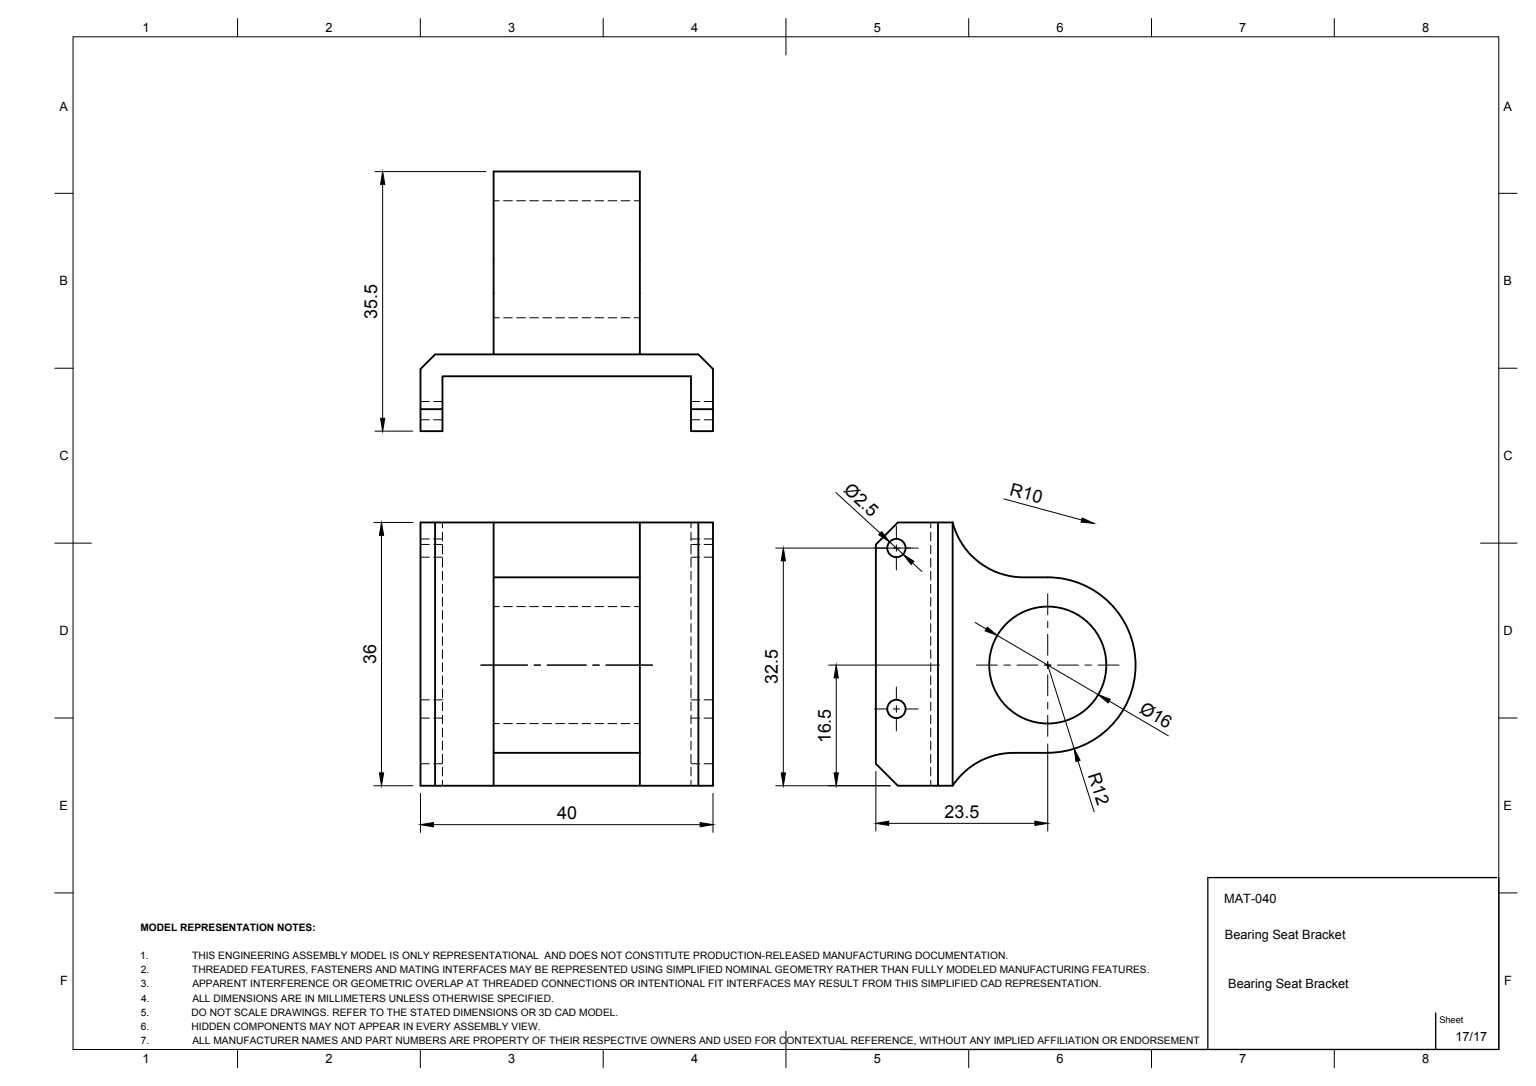
ISO-10303-21;
HEADER;
/* Generated by software containing ST-Developer
 * from STEP Tools, Inc. (www.steptools.com) 
 */

FILE_DESCRIPTION(
/* description */ ('STEP AP214'),
/* implementation_level */ '2;1');

FILE_NAME(
/* name */ 'Bearing Seat Bracket.step',
/* time_stamp */ '2026-11-14T21:53:28-08:00',
/* author */ (''),
/* organization */ (''),
/* preprocessor_version */ 'ST-DEVELOPER v20.2',
/* originating_system */ 'Autodesk Translation Framework v15.17.0.0',
/* authorisation */ '');

FILE_SCHEMA (('AUTOMOTIVE_DESIGN { 1 0 10303 214 3 1 1 }'));
ENDSEC;

DATA;
#10=MECHANICAL_DESIGN_GEOMETRIC_PRESENTATION_REPRESENTATION('',(#332),#20176);
#300=SHAPE_REPRESENTATION_RELATIONSHIP('SRR','None',#20264,#312);
#312=ADVANCED_BREP_SHAPE_REPRESENTATION('',(#359),#20170);
#332=STYLED_ITEM('',(#20338),#359);
#359=MANIFOLD_SOLID_BREP('Body1',#10950);
#546=FACE_BOUND('',#2149,.T.);
#547=FACE_BOUND('',#2150,.T.);
#548=FACE_BOUND('',#2153,.T.);
#549=FACE_BOUND('',#2154,.T.);
#550=FACE_BOUND('',#2157,.T.);
#551=FACE_BOUND('',#2158,.T.);
#552=FACE_BOUND('',#2160,.T.);
#553=FACE_BOUND('',#2161,.T.);
#554=FACE_BOUND('',#2174,.T.);
#555=FACE_BOUND('',#2177,.T.);
#846=PLANE('',#11980);
#847=PLANE('',#11981);
#848=PLANE('',#11982);
#849=PLANE('',#11983);
#850=PLANE('',#11984);
#851=PLANE('',#11985);
#852=PLANE('',#11986);
#853=PLANE('',#11987);
#854=PLANE('',#11988);
#855=PLANE('',#11989);
#856=PLANE('',#11990);
#857=PLANE('',#11991);
#858=PLANE('',#11992);
#859=PLANE('',#11996);
#860=PLANE('',#11997);
#861=PLANE('',#12004);
#862=PLANE('',#12005);
#863=PLANE('',#12006);
#864=PLANE('',#12007);
#865=PLANE('',#12008);
#866=PLANE('',#12009);
#1384=FACE_OUTER_BOUND('',#2142,.T.);
#1385=FACE_OUTER_BOUND('',#2143,.T.);
#1386=FACE_OUTER_BOUND('',#2144,.T.);
#1387=FACE_OUTER_BOUND('',#2145,.T.);
#1388=FACE_OUTER_BOUND('',#2146,.T.);
#1389=FACE_OUTER_BOUND('',#2147,.T.);
#1390=FACE_OUTER_BOUND('',#2148,.T.);
#1391=FACE_OUTER_BOUND('',#2151,.T.);
#1392=FACE_OUTER_BOUND('',#2152,.T.);
#1393=FACE_OUTER_BOUND('',#2155,.T.);
#1394=FACE_OUTER_BOUND('',#2156,.T.);
#1395=FACE_OUTER_BOUND('',#2159,.T.);
#1396=FACE_OUTER_BOUND('',#2162,.T.);
#1397=FACE_OUTER_BOUND('',#2163,.T.);
#1398=FACE_OUTER_BOUND('',#2164,.T.);
#1399=FACE_OUTER_BOUND('',#2165,.T.);
#1400=FACE_OUTER_BOUND('',#2166,.T.);
#1401=FACE_OUTER_BOUND('',#2167,.T.);
#1402=FACE_OUTER_BOUND('',#2168,.T.);
#1403=FACE_OUTER_BOUND('',#2169,.T.);
#1404=FACE_OUTER_BOUND('',#2170,.T.);
#1405=FACE_OUTER_BOUND('',#2171,.T.);
#1406=FACE_OUTER_BOUND('',#2172,.T.);
#1407=FACE_OUTER_BOUND('',#2173,.T.);
#1408=FACE_OUTER_BOUND('',#2175,.T.);
#1409=FACE_OUTER_BOUND('',#2176,.T.);
#1410=FACE_OUTER_BOUND('',#2178,.T.);
#1411=FACE_OUTER_BOUND('',#2179,.T.);
#1412=FACE_OUTER_BOUND('',#2180,.T.);
#2142=EDGE_LOOP('',(#9717,#9718,#9719,#9720));
#2143=EDGE_LOOP('',(#9721,#9722,#9723,#9724));
#2144=EDGE_LOOP('',(#9725,#9726,#9727,#9728));
#2145=EDGE_LOOP('',(#9729,#9730,#9731,#9732));
#2146=EDGE_LOOP('',(#9733,#9734,#9735,#9736));
#2147=EDGE_LOOP('',(#9737,#9738,#9739,#9740));
#2148=EDGE_LOOP('',(#9741,#9742,#9743,#9744,#9745,#9746));
#2149=EDGE_LOOP('',(#9747));
#2150=EDGE_LOOP('',(#9748));
#2151=EDGE_LOOP('',(#9749,#9750,#9751,#9752));
#2152=EDGE_LOOP('',(#9753,#9754,#9755,#9756,#9757,#9758));
#2153=EDGE_LOOP('',(#9759));
#2154=EDGE_LOOP('',(#9760));
#2155=EDGE_LOOP('',(#9761,#9762,#9763,#9764));
#2156=EDGE_LOOP('',(#9765,#9766,#9767,#9768,#9769,#9770));
#2157=EDGE_LOOP('',(#9771));
#2158=EDGE_LOOP('',(#9772));
#2159=EDGE_LOOP('',(#9773,#9774,#9775,#9776,#9777,#9778));
#2160=EDGE_LOOP('',(#9779));
#2161=EDGE_LOOP('',(#9780));
#2162=EDGE_LOOP('',(#9781,#9782,#9783,#9784,#9785,#9786,#9787,#9788,#9789,
#9790,#9791,#9792));
#2163=EDGE_LOOP('',(#9793,#9794,#9795,#9796,#9797,#9798,#9799,#9800,#9801,
#9802,#9803,#9804));
#2164=EDGE_LOOP('',(#9805,#9806,#9807,#9808));
#2165=EDGE_LOOP('',(#9809,#9810,#9811,#9812));
#2166=EDGE_LOOP('',(#9813,#9814,#9815,#9816));
#2167=EDGE_LOOP('',(#9817,#9818,#9819,#9820));
#2168=EDGE_LOOP('',(#9821,#9822,#9823,#9824));
#2169=EDGE_LOOP('',(#9825,#9826,#9827,#9828));
#2170=EDGE_LOOP('',(#9829,#9830,#9831,#9832));
#2171=EDGE_LOOP('',(#9833,#9834,#9835,#9836));
#2172=EDGE_LOOP('',(#9837,#9838,#9839,#9840));
#2173=EDGE_LOOP('',(#9841,#9842,#9843,#9844,#9845,#9846));
#2174=EDGE_LOOP('',(#9847));
#2175=EDGE_LOOP('',(#9848,#9849,#9850,#9851));
#2176=EDGE_LOOP('',(#9852,#9853,#9854,#9855,#9856,#9857));
#2177=EDGE_LOOP('',(#9858));
#2178=EDGE_LOOP('',(#9859,#9860,#9861,#9862));
#2179=EDGE_LOOP('',(#9863,#9864,#9865,#9866));
#2180=EDGE_LOOP('',(#9867,#9868,#9869,#9870));
#3146=LINE('',#19626,#4134);
#3147=LINE('',#19632,#4135);
#3148=LINE('',#19638,#4136);
#3149=LINE('',#19644,#4137);
#3150=LINE('',#19650,#4138);
#3151=LINE('',#19655,#4139);
#3152=LINE('',#19657,#4140);
#3153=LINE('',#19659,#4141);
#3154=LINE('',#19660,#4142);
#3155=LINE('',#19664,#4143);
#3156=LINE('',#19665,#4144);
#3157=LINE('',#19667,#4145);
#3158=LINE('',#19669,#4146);
#3159=LINE('',#19670,#4147);
#3160=LINE('',#19673,#4148);
#3161=LINE('',#19675,#4149);
#3162=LINE('',#19676,#4150);
#3163=LINE('',#19680,#4151);
#3164=LINE('',#19682,#4152);
#3165=LINE('',#19683,#4153);
#3166=LINE('',#19685,#4154);
#3167=LINE('',#19686,#4155);
#3168=LINE('',#19690,#4156);
#3169=LINE('',#19691,#4157);
#3170=LINE('',#19692,#4158);
#3171=LINE('',#19696,#4159);
#3172=LINE('',#19698,#4160);
#3173=LINE('',#19700,#4161);
#3174=LINE('',#19701,#4162);
#3175=LINE('',#19702,#4163);
#3176=LINE('',#19706,#4164);
#3177=LINE('',#19708,#4165);
#3178=LINE('',#19710,#4166);
#3179=LINE('',#19711,#4167);
#3180=LINE('',#19712,#4168);
#3181=LINE('',#19715,#4169);
#3182=LINE('',#19717,#4170);
#3183=LINE('',#19719,#4171);
#3184=LINE('',#19721,#4172);
#3185=LINE('',#19722,#4173);
#3186=LINE('',#19723,#4174);
#3187=LINE('',#19724,#4175);
#3188=LINE('',#19728,#4176);
#3189=LINE('',#19729,#4177);
#3190=LINE('',#19730,#4178);
#3191=LINE('',#19731,#4179);
#3192=LINE('',#19733,#4180);
#3193=LINE('',#19735,#4181);
#3194=LINE('',#19736,#4182);
#3195=LINE('',#19746,#4183);
#3196=LINE('',#19749,#4184);
#3197=LINE('',#19752,#4185);
#3198=LINE('',#19754,#4186);
#3199=LINE('',#19755,#4187);
#3200=LINE('',#19758,#4188);
#3201=LINE('',#19760,#4189);
#3202=LINE('',#19761,#4190);
#3203=LINE('',#19769,#4191);
#3204=LINE('',#19771,#4192);
#3205=LINE('',#19773,#4193);
#3206=LINE('',#19775,#4194);
#4134=VECTOR('',#14806,8.);
#4135=VECTOR('',#14813,1.25);
#4136=VECTOR('',#14820,1.25);
#4137=VECTOR('',#14827,1.25);
#4138=VECTOR('',#14834,1.25);
#4139=VECTOR('',#14839,1000.);
#4140=VECTOR('',#14840,1000.);
#4141=VECTOR('',#14841,1000.);
#4142=VECTOR('',#14842,1000.);
#4143=VECTOR('',#14845,1000.);
#4144=VECTOR('',#14846,1000.);
#4145=VECTOR('',#14847,1000.);
#4146=VECTOR('',#14848,1000.);
#4147=VECTOR('',#14849,1000.);
#4148=VECTOR('',#14852,1000.);
#4149=VECTOR('',#14853,1000.);
#4150=VECTOR('',#14854,1000.);
#4151=VECTOR('',#14857,1000.);
#4152=VECTOR('',#14858,1000.);
#4153=VECTOR('',#14859,1000.);
#4154=VECTOR('',#14860,1000.);
#4155=VECTOR('',#14861,1000.);
#4156=VECTOR('',#14864,1000.);
#4157=VECTOR('',#14865,1000.);
#4158=VECTOR('',#14866,1000.);
#4159=VECTOR('',#14869,1000.);
#4160=VECTOR('',#14870,1000.);
#4161=VECTOR('',#14871,1000.);
#4162=VECTOR('',#14872,1000.);
#4163=VECTOR('',#14873,1000.);
#4164=VECTOR('',#14876,1000.);
#4165=VECTOR('',#14877,1000.);
#4166=VECTOR('',#14878,1000.);
#4167=VECTOR('',#14879,1000.);
#4168=VECTOR('',#14880,1000.);
#4169=VECTOR('',#14883,1000.);
#4170=VECTOR('',#14884,1000.);
#4171=VECTOR('',#14885,1000.);
#4172=VECTOR('',#14886,1000.);
#4173=VECTOR('',#14887,1000.);
#4174=VECTOR('',#14888,1000.);
#4175=VECTOR('',#14889,1000.);
#4176=VECTOR('',#14892,1000.);
#4177=VECTOR('',#14893,1000.);
#4178=VECTOR('',#14894,1000.);
#4179=VECTOR('',#14895,1000.);
#4180=VECTOR('',#14896,1000.);
#4181=VECTOR('',#14897,1000.);
#4182=VECTOR('',#14898,1000.);
#4183=VECTOR('',#14911,1000.);
#4184=VECTOR('',#14914,1000.);
#4185=VECTOR('',#14917,1000.);
#4186=VECTOR('',#14918,1000.);
#4187=VECTOR('',#14919,1000.);
#4188=VECTOR('',#14922,1000.);
#4189=VECTOR('',#14923,1000.);
#4190=VECTOR('',#14924,1000.);
#4191=VECTOR('',#14939,1000.);
#4192=VECTOR('',#14942,1000.);
#4193=VECTOR('',#14945,1000.);
#4194=VECTOR('',#14948,1000.);
#4635=CIRCLE('',#11966,8.);
#4636=CIRCLE('',#11967,8.00000000000001);
#4637=CIRCLE('',#11969,1.25);
#4638=CIRCLE('',#11970,1.25);
#4639=CIRCLE('',#11972,1.25);
#4640=CIRCLE('',#11973,1.25);
#4641=CIRCLE('',#11975,1.25);
#4642=CIRCLE('',#11976,1.25);
#4643=CIRCLE('',#11978,1.25);
#4644=CIRCLE('',#11979,1.25);
#4645=CIRCLE('',#11994,12.);
#4646=CIRCLE('',#11995,12.);
#4647=CIRCLE('',#11999,10.);
#4648=CIRCLE('',#12000,10.);
#4649=CIRCLE('',#12002,10.);
#4650=CIRCLE('',#12003,10.);
#5542=VERTEX_POINT('',#19623);
#5543=VERTEX_POINT('',#19625);
#5544=VERTEX_POINT('',#19629);
#5545=VERTEX_POINT('',#19631);
#5546=VERTEX_POINT('',#19635);
#5547=VERTEX_POINT('',#19637);
#5548=VERTEX_POINT('',#19641);
#5549=VERTEX_POINT('',#19643);
#5550=VERTEX_POINT('',#19647);
#5551=VERTEX_POINT('',#19649);
#5552=VERTEX_POINT('',#19653);
#5553=VERTEX_POINT('',#19654);
#5554=VERTEX_POINT('',#19656);
#5555=VERTEX_POINT('',#19658);
#5556=VERTEX_POINT('',#19662);
#5557=VERTEX_POINT('',#19663);
#5558=VERTEX_POINT('',#19666);
#5559=VERTEX_POINT('',#19668);
#5560=VERTEX_POINT('',#19672);
#5561=VERTEX_POINT('',#19674);
#5562=VERTEX_POINT('',#19678);
#5563=VERTEX_POINT('',#19679);
#5564=VERTEX_POINT('',#19681);
#5565=VERTEX_POINT('',#19684);
#5566=VERTEX_POINT('',#19688);
#5567=VERTEX_POINT('',#19689);
#5568=VERTEX_POINT('',#19694);
#5569=VERTEX_POINT('',#19695);
#5570=VERTEX_POINT('',#19697);
#5571=VERTEX_POINT('',#19699);
#5572=VERTEX_POINT('',#19704);
#5573=VERTEX_POINT('',#19705);
#5574=VERTEX_POINT('',#19707);
#5575=VERTEX_POINT('',#19709);
#5576=VERTEX_POINT('',#19714);
#5577=VERTEX_POINT('',#19716);
#5578=VERTEX_POINT('',#19718);
#5579=VERTEX_POINT('',#19720);
#5580=VERTEX_POINT('',#19726);
#5581=VERTEX_POINT('',#19727);
#5582=VERTEX_POINT('',#19732);
#5583=VERTEX_POINT('',#19734);
#5584=VERTEX_POINT('',#19742);
#5585=VERTEX_POINT('',#19743);
#5586=VERTEX_POINT('',#19745);
#5587=VERTEX_POINT('',#19747);
#5588=VERTEX_POINT('',#19751);
#5589=VERTEX_POINT('',#19753);
#5590=VERTEX_POINT('',#19757);
#5591=VERTEX_POINT('',#19759);
#6969=EDGE_CURVE('',#5542,#5542,#4635,.T.);
#6970=EDGE_CURVE('',#5542,#5543,#3146,.T.);
#6971=EDGE_CURVE('',#5543,#5543,#4636,.T.);
#6972=EDGE_CURVE('',#5544,#5544,#4637,.T.);
#6973=EDGE_CURVE('',#5544,#5545,#3147,.T.);
#6974=EDGE_CURVE('',#5545,#5545,#4638,.T.);
#6975=EDGE_CURVE('',#5546,#5546,#4639,.T.);
#6976=EDGE_CURVE('',#5546,#5547,#3148,.T.);
#6977=EDGE_CURVE('',#5547,#5547,#4640,.T.);
#6978=EDGE_CURVE('',#5548,#5548,#4641,.T.);
#6979=EDGE_CURVE('',#5548,#5549,#3149,.T.);
#6980=EDGE_CURVE('',#5549,#5549,#4642,.T.);
#6981=EDGE_CURVE('',#5550,#5550,#4643,.T.);
#6982=EDGE_CURVE('',#5550,#5551,#3150,.T.);
#6983=EDGE_CURVE('',#5551,#5551,#4644,.T.);
#6984=EDGE_CURVE('',#5552,#5553,#3151,.T.);
#6985=EDGE_CURVE('',#5552,#5554,#3152,.T.);
#6986=EDGE_CURVE('',#5554,#5555,#3153,.T.);
#6987=EDGE_CURVE('',#5555,#5553,#3154,.T.);
#6988=EDGE_CURVE('',#5556,#5557,#3155,.T.);
#6989=EDGE_CURVE('',#5556,#5552,#3156,.T.);
#6990=EDGE_CURVE('',#5553,#5558,#3157,.T.);
#6991=EDGE_CURVE('',#5558,#5559,#3158,.T.);
#6992=EDGE_CURVE('',#5557,#5559,#3159,.T.);
#6993=EDGE_CURVE('',#5559,#5560,#3160,.T.);
#6994=EDGE_CURVE('',#5561,#5560,#3161,.T.);
#6995=EDGE_CURVE('',#5557,#5561,#3162,.T.);
#6996=EDGE_CURVE('',#5562,#5563,#3163,.T.);
#6997=EDGE_CURVE('',#5562,#5564,#3164,.T.);
#6998=EDGE_CURVE('',#5561,#5564,#3165,.T.);
#6999=EDGE_CURVE('',#5560,#5565,#3166,.T.);
#7000=EDGE_CURVE('',#5565,#5563,#3167,.T.);
#7001=EDGE_CURVE('',#5566,#5567,#3168,.T.);
#7002=EDGE_CURVE('',#5566,#5562,#3169,.T.);
#7003=EDGE_CURVE('',#5563,#5567,#3170,.T.);
#7004=EDGE_CURVE('',#5568,#5569,#3171,.T.);
#7005=EDGE_CURVE('',#5569,#5570,#3172,.T.);
#7006=EDGE_CURVE('',#5571,#5570,#3173,.T.);
#7007=EDGE_CURVE('',#5571,#5566,#3174,.T.);
#7008=EDGE_CURVE('',#5567,#5568,#3175,.T.);
#7009=EDGE_CURVE('',#5572,#5573,#3176,.T.);
#7010=EDGE_CURVE('',#5572,#5574,#3177,.T.);
#7011=EDGE_CURVE('',#5574,#5575,#3178,.T.);
#7012=EDGE_CURVE('',#5575,#5555,#3179,.T.);
#7013=EDGE_CURVE('',#5554,#5573,#3180,.T.);
#7014=EDGE_CURVE('',#5570,#5576,#3181,.T.);
#7015=EDGE_CURVE('',#5576,#5577,#3182,.T.);
#7016=EDGE_CURVE('',#5577,#5578,#3183,.T.);
#7017=EDGE_CURVE('',#5579,#5578,#3184,.T.);
#7018=EDGE_CURVE('',#5579,#5572,#3185,.T.);
#7019=EDGE_CURVE('',#5573,#5556,#3186,.T.);
#7020=EDGE_CURVE('',#5564,#5571,#3187,.T.);
#7021=EDGE_CURVE('',#5580,#5581,#3188,.T.);
#7022=EDGE_CURVE('',#5580,#5569,#3189,.T.);
#7023=EDGE_CURVE('',#5568,#5565,#3190,.T.);
#7024=EDGE_CURVE('',#5558,#5575,#3191,.T.);
#7025=EDGE_CURVE('',#5574,#5582,#3192,.T.);
#7026=EDGE_CURVE('',#5582,#5583,#3193,.T.);
#7027=EDGE_CURVE('',#5581,#5583,#3194,.T.);
#7028=EDGE_CURVE('',#5584,#5585,#4645,.T.);
#7029=EDGE_CURVE('',#5584,#5586,#3195,.T.);
#7030=EDGE_CURVE('',#5587,#5586,#4646,.T.);
#7031=EDGE_CURVE('',#5585,#5587,#3196,.T.);
#7032=EDGE_CURVE('',#5585,#5588,#3197,.T.);
#7033=EDGE_CURVE('',#5589,#5587,#3198,.T.);
#7034=EDGE_CURVE('',#5589,#5588,#3199,.T.);
#7035=EDGE_CURVE('',#5590,#5584,#3200,.T.);
#7036=EDGE_CURVE('',#5590,#5591,#3201,.T.);
#7037=EDGE_CURVE('',#5586,#5591,#3202,.T.);
#7038=EDGE_CURVE('',#5590,#5581,#4647,.T.);
#7039=EDGE_CURVE('',#5583,#5591,#4648,.T.);
#7040=EDGE_CURVE('',#5577,#5588,#4649,.T.);
#7041=EDGE_CURVE('',#5589,#5578,#4650,.T.);
#7042=EDGE_CURVE('',#5583,#5578,#3203,.T.);
#7043=EDGE_CURVE('',#5582,#5579,#3204,.T.);
#7044=EDGE_CURVE('',#5581,#5577,#3205,.T.);
#7045=EDGE_CURVE('',#5576,#5580,#3206,.T.);
#9717=ORIENTED_EDGE('',*,*,#6969,.T.);
#9718=ORIENTED_EDGE('',*,*,#6970,.T.);
#9719=ORIENTED_EDGE('',*,*,#6971,.T.);
#9720=ORIENTED_EDGE('',*,*,#6970,.F.);
#9721=ORIENTED_EDGE('',*,*,#6972,.F.);
#9722=ORIENTED_EDGE('',*,*,#6973,.T.);
#9723=ORIENTED_EDGE('',*,*,#6974,.F.);
#9724=ORIENTED_EDGE('',*,*,#6973,.F.);
#9725=ORIENTED_EDGE('',*,*,#6975,.F.);
#9726=ORIENTED_EDGE('',*,*,#6976,.T.);
#9727=ORIENTED_EDGE('',*,*,#6977,.T.);
#9728=ORIENTED_EDGE('',*,*,#6976,.F.);
#9729=ORIENTED_EDGE('',*,*,#6978,.F.);
#9730=ORIENTED_EDGE('',*,*,#6979,.T.);
#9731=ORIENTED_EDGE('',*,*,#6980,.F.);
#9732=ORIENTED_EDGE('',*,*,#6979,.F.);
#9733=ORIENTED_EDGE('',*,*,#6981,.F.);
#9734=ORIENTED_EDGE('',*,*,#6982,.T.);
#9735=ORIENTED_EDGE('',*,*,#6983,.T.);
#9736=ORIENTED_EDGE('',*,*,#6982,.F.);
#9737=ORIENTED_EDGE('',*,*,#6984,.F.);
#9738=ORIENTED_EDGE('',*,*,#6985,.T.);
#9739=ORIENTED_EDGE('',*,*,#6986,.T.);
#9740=ORIENTED_EDGE('',*,*,#6987,.T.);
#9741=ORIENTED_EDGE('',*,*,#6988,.F.);
#9742=ORIENTED_EDGE('',*,*,#6989,.T.);
#9743=ORIENTED_EDGE('',*,*,#6984,.T.);
#9744=ORIENTED_EDGE('',*,*,#6990,.T.);
#9745=ORIENTED_EDGE('',*,*,#6991,.T.);
#9746=ORIENTED_EDGE('',*,*,#6992,.F.);
#9747=ORIENTED_EDGE('',*,*,#6975,.T.);
#9748=ORIENTED_EDGE('',*,*,#6981,.T.);
#9749=ORIENTED_EDGE('',*,*,#6993,.T.);
#9750=ORIENTED_EDGE('',*,*,#6994,.F.);
#9751=ORIENTED_EDGE('',*,*,#6995,.F.);
#9752=ORIENTED_EDGE('',*,*,#6992,.T.);
#9753=ORIENTED_EDGE('',*,*,#6996,.F.);
#9754=ORIENTED_EDGE('',*,*,#6997,.T.);
#9755=ORIENTED_EDGE('',*,*,#6998,.F.);
#9756=ORIENTED_EDGE('',*,*,#6994,.T.);
#9757=ORIENTED_EDGE('',*,*,#6999,.T.);
#9758=ORIENTED_EDGE('',*,*,#7000,.T.);
#9759=ORIENTED_EDGE('',*,*,#6974,.T.);
#9760=ORIENTED_EDGE('',*,*,#6980,.T.);
#9761=ORIENTED_EDGE('',*,*,#7001,.F.);
#9762=ORIENTED_EDGE('',*,*,#7002,.T.);
#9763=ORIENTED_EDGE('',*,*,#6996,.T.);
#9764=ORIENTED_EDGE('',*,*,#7003,.T.);
#9765=ORIENTED_EDGE('',*,*,#7004,.T.);
#9766=ORIENTED_EDGE('',*,*,#7005,.T.);
#9767=ORIENTED_EDGE('',*,*,#7006,.F.);
#9768=ORIENTED_EDGE('',*,*,#7007,.T.);
#9769=ORIENTED_EDGE('',*,*,#7001,.T.);
#9770=ORIENTED_EDGE('',*,*,#7008,.T.);
#9771=ORIENTED_EDGE('',*,*,#6972,.T.);
#9772=ORIENTED_EDGE('',*,*,#6978,.T.);
#9773=ORIENTED_EDGE('',*,*,#7009,.F.);
#9774=ORIENTED_EDGE('',*,*,#7010,.T.);
#9775=ORIENTED_EDGE('',*,*,#7011,.T.);
#9776=ORIENTED_EDGE('',*,*,#7012,.T.);
#9777=ORIENTED_EDGE('',*,*,#6986,.F.);
#9778=ORIENTED_EDGE('',*,*,#7013,.T.);
#9779=ORIENTED_EDGE('',*,*,#6977,.F.);
#9780=ORIENTED_EDGE('',*,*,#6983,.F.);
#9781=ORIENTED_EDGE('',*,*,#7006,.T.);
#9782=ORIENTED_EDGE('',*,*,#7014,.T.);
#9783=ORIENTED_EDGE('',*,*,#7015,.T.);
#9784=ORIENTED_EDGE('',*,*,#7016,.T.);
#9785=ORIENTED_EDGE('',*,*,#7017,.F.);
#9786=ORIENTED_EDGE('',*,*,#7018,.T.);
#9787=ORIENTED_EDGE('',*,*,#7009,.T.);
#9788=ORIENTED_EDGE('',*,*,#7019,.T.);
#9789=ORIENTED_EDGE('',*,*,#6988,.T.);
#9790=ORIENTED_EDGE('',*,*,#6995,.T.);
#9791=ORIENTED_EDGE('',*,*,#6998,.T.);
#9792=ORIENTED_EDGE('',*,*,#7020,.T.);
#9793=ORIENTED_EDGE('',*,*,#7021,.F.);
#9794=ORIENTED_EDGE('',*,*,#7022,.T.);
#9795=ORIENTED_EDGE('',*,*,#7004,.F.);
#9796=ORIENTED_EDGE('',*,*,#7023,.T.);
#9797=ORIENTED_EDGE('',*,*,#6999,.F.);
#9798=ORIENTED_EDGE('',*,*,#6993,.F.);
#9799=ORIENTED_EDGE('',*,*,#6991,.F.);
#9800=ORIENTED_EDGE('',*,*,#7024,.T.);
#9801=ORIENTED_EDGE('',*,*,#7011,.F.);
#9802=ORIENTED_EDGE('',*,*,#7025,.T.);
#9803=ORIENTED_EDGE('',*,*,#7026,.T.);
#9804=ORIENTED_EDGE('',*,*,#7027,.F.);
#9805=ORIENTED_EDGE('',*,*,#6997,.F.);
#9806=ORIENTED_EDGE('',*,*,#7002,.F.);
#9807=ORIENTED_EDGE('',*,*,#7007,.F.);
#9808=ORIENTED_EDGE('',*,*,#7020,.F.);
#9809=ORIENTED_EDGE('',*,*,#7000,.F.);
#9810=ORIENTED_EDGE('',*,*,#7023,.F.);
#9811=ORIENTED_EDGE('',*,*,#7008,.F.);
#9812=ORIENTED_EDGE('',*,*,#7003,.F.);
#9813=ORIENTED_EDGE('',*,*,#7013,.F.);
#9814=ORIENTED_EDGE('',*,*,#6985,.F.);
#9815=ORIENTED_EDGE('',*,*,#6989,.F.);
#9816=ORIENTED_EDGE('',*,*,#7019,.F.);
#9817=ORIENTED_EDGE('',*,*,#7012,.F.);
#9818=ORIENTED_EDGE('',*,*,#7024,.F.);
#9819=ORIENTED_EDGE('',*,*,#6990,.F.);
#9820=ORIENTED_EDGE('',*,*,#6987,.F.);
#9821=ORIENTED_EDGE('',*,*,#7028,.F.);
#9822=ORIENTED_EDGE('',*,*,#7029,.T.);
#9823=ORIENTED_EDGE('',*,*,#7030,.F.);
#9824=ORIENTED_EDGE('',*,*,#7031,.F.);
#9825=ORIENTED_EDGE('',*,*,#7032,.F.);
#9826=ORIENTED_EDGE('',*,*,#7031,.T.);
#9827=ORIENTED_EDGE('',*,*,#7033,.F.);
#9828=ORIENTED_EDGE('',*,*,#7034,.T.);
#9829=ORIENTED_EDGE('',*,*,#7035,.F.);
#9830=ORIENTED_EDGE('',*,*,#7036,.T.);
#9831=ORIENTED_EDGE('',*,*,#7037,.F.);
#9832=ORIENTED_EDGE('',*,*,#7029,.F.);
#9833=ORIENTED_EDGE('',*,*,#7036,.F.);
#9834=ORIENTED_EDGE('',*,*,#7038,.T.);
#9835=ORIENTED_EDGE('',*,*,#7027,.T.);
#9836=ORIENTED_EDGE('',*,*,#7039,.T.);
#9837=ORIENTED_EDGE('',*,*,#7016,.F.);
#9838=ORIENTED_EDGE('',*,*,#7040,.T.);
#9839=ORIENTED_EDGE('',*,*,#7034,.F.);
#9840=ORIENTED_EDGE('',*,*,#7041,.T.);
#9841=ORIENTED_EDGE('',*,*,#7042,.T.);
#9842=ORIENTED_EDGE('',*,*,#7041,.F.);
#9843=ORIENTED_EDGE('',*,*,#7033,.T.);
#9844=ORIENTED_EDGE('',*,*,#7030,.T.);
#9845=ORIENTED_EDGE('',*,*,#7037,.T.);
#9846=ORIENTED_EDGE('',*,*,#7039,.F.);
#9847=ORIENTED_EDGE('',*,*,#6971,.F.);
#9848=ORIENTED_EDGE('',*,*,#7026,.F.);
#9849=ORIENTED_EDGE('',*,*,#7043,.T.);
#9850=ORIENTED_EDGE('',*,*,#7017,.T.);
#9851=ORIENTED_EDGE('',*,*,#7042,.F.);
#9852=ORIENTED_EDGE('',*,*,#7035,.T.);
#9853=ORIENTED_EDGE('',*,*,#7028,.T.);
#9854=ORIENTED_EDGE('',*,*,#7032,.T.);
#9855=ORIENTED_EDGE('',*,*,#7040,.F.);
#9856=ORIENTED_EDGE('',*,*,#7044,.F.);
#9857=ORIENTED_EDGE('',*,*,#7038,.F.);
#9858=ORIENTED_EDGE('',*,*,#6969,.F.);
#9859=ORIENTED_EDGE('',*,*,#7015,.F.);
#9860=ORIENTED_EDGE('',*,*,#7045,.T.);
#9861=ORIENTED_EDGE('',*,*,#7021,.T.);
#9862=ORIENTED_EDGE('',*,*,#7044,.T.);
#9863=ORIENTED_EDGE('',*,*,#7022,.F.);
#9864=ORIENTED_EDGE('',*,*,#7045,.F.);
#9865=ORIENTED_EDGE('',*,*,#7014,.F.);
#9866=ORIENTED_EDGE('',*,*,#7005,.F.);
#9867=ORIENTED_EDGE('',*,*,#7025,.F.);
#9868=ORIENTED_EDGE('',*,*,#7010,.F.);
#9869=ORIENTED_EDGE('',*,*,#7018,.F.);
#9870=ORIENTED_EDGE('',*,*,#7043,.F.);
#10321=CYLINDRICAL_SURFACE('',#11965,8.);
#10322=CYLINDRICAL_SURFACE('',#11968,1.25);
#10323=CYLINDRICAL_SURFACE('',#11971,1.25);
#10324=CYLINDRICAL_SURFACE('',#11974,1.25);
#10325=CYLINDRICAL_SURFACE('',#11977,1.25);
#10326=CYLINDRICAL_SURFACE('',#11993,12.);
#10327=CYLINDRICAL_SURFACE('',#11998,10.);
#10328=CYLINDRICAL_SURFACE('',#12001,10.);
#10836=ADVANCED_FACE('',(#1384),#10321,.F.);
#10837=ADVANCED_FACE('',(#1385),#10322,.F.);
#10838=ADVANCED_FACE('',(#1386),#10323,.F.);
#10839=ADVANCED_FACE('',(#1387),#10324,.F.);
#10840=ADVANCED_FACE('',(#1388),#10325,.F.);
#10841=ADVANCED_FACE('',(#1389),#846,.F.);
#10842=ADVANCED_FACE('',(#1390,#546,#547),#847,.F.);
#10843=ADVANCED_FACE('',(#1391),#848,.F.);
#10844=ADVANCED_FACE('',(#1392,#548,#549),#849,.F.);
#10845=ADVANCED_FACE('',(#1393),#850,.F.);
#10846=ADVANCED_FACE('',(#1394,#550,#551),#851,.F.);
#10847=ADVANCED_FACE('',(#1395,#552,#553),#852,.F.);
#10848=ADVANCED_FACE('',(#1396),#853,.T.);
#10849=ADVANCED_FACE('',(#1397),#854,.F.);
#10850=ADVANCED_FACE('',(#1398),#855,.T.);
#10851=ADVANCED_FACE('',(#1399),#856,.F.);
#10852=ADVANCED_FACE('',(#1400),#857,.T.);
#10853=ADVANCED_FACE('',(#1401),#858,.F.);
#10854=ADVANCED_FACE('',(#1402),#10326,.T.);
#10855=ADVANCED_FACE('',(#1403),#859,.T.);
#10856=ADVANCED_FACE('',(#1404),#860,.T.);
#10857=ADVANCED_FACE('',(#1405),#10327,.F.);
#10858=ADVANCED_FACE('',(#1406),#10328,.F.);
#10859=ADVANCED_FACE('',(#1407,#554),#861,.F.);
#10860=ADVANCED_FACE('',(#1408),#862,.F.);
#10861=ADVANCED_FACE('',(#1409,#555),#863,.F.);
#10862=ADVANCED_FACE('',(#1410),#864,.F.);
#10863=ADVANCED_FACE('',(#1411),#865,.F.);
#10864=ADVANCED_FACE('',(#1412),#866,.F.);
#10950=CLOSED_SHELL('',(#10836,#10837,#10838,#10839,#10840,#10841,#10842,
#10843,#10844,#10845,#10846,#10847,#10848,#10849,#10850,#10851,#10852,#10853,
#10854,#10855,#10856,#10857,#10858,#10859,#10860,#10861,#10862,#10863,#10864));
#11964=AXIS2_PLACEMENT_3D('',#19621,#14800,#14801);
#11965=AXIS2_PLACEMENT_3D('',#19622,#14802,#14803);
#11966=AXIS2_PLACEMENT_3D('',#19624,#14804,#14805);
#11967=AXIS2_PLACEMENT_3D('',#19627,#14807,#14808);
#11968=AXIS2_PLACEMENT_3D('',#19628,#14809,#14810);
#11969=AXIS2_PLACEMENT_3D('',#19630,#14811,#14812);
#11970=AXIS2_PLACEMENT_3D('',#19633,#14814,#14815);
#11971=AXIS2_PLACEMENT_3D('',#19634,#14816,#14817);
#11972=AXIS2_PLACEMENT_3D('',#19636,#14818,#14819);
#11973=AXIS2_PLACEMENT_3D('',#19639,#14821,#14822);
#11974=AXIS2_PLACEMENT_3D('',#19640,#14823,#14824);
#11975=AXIS2_PLACEMENT_3D('',#19642,#14825,#14826);
#11976=AXIS2_PLACEMENT_3D('',#19645,#14828,#14829);
#11977=AXIS2_PLACEMENT_3D('',#19646,#14830,#14831);
#11978=AXIS2_PLACEMENT_3D('',#19648,#14832,#14833);
#11979=AXIS2_PLACEMENT_3D('',#19651,#14835,#14836);
#11980=AXIS2_PLACEMENT_3D('',#19652,#14837,#14838);
#11981=AXIS2_PLACEMENT_3D('',#19661,#14843,#14844);
#11982=AXIS2_PLACEMENT_3D('',#19671,#14850,#14851);
#11983=AXIS2_PLACEMENT_3D('',#19677,#14855,#14856);
#11984=AXIS2_PLACEMENT_3D('',#19687,#14862,#14863);
#11985=AXIS2_PLACEMENT_3D('',#19693,#14867,#14868);
#11986=AXIS2_PLACEMENT_3D('',#19703,#14874,#14875);
#11987=AXIS2_PLACEMENT_3D('',#19713,#14881,#14882);
#11988=AXIS2_PLACEMENT_3D('',#19725,#14890,#14891);
#11989=AXIS2_PLACEMENT_3D('',#19737,#14899,#14900);
#11990=AXIS2_PLACEMENT_3D('',#19738,#14901,#14902);
#11991=AXIS2_PLACEMENT_3D('',#19739,#14903,#14904);
#11992=AXIS2_PLACEMENT_3D('',#19740,#14905,#14906);
#11993=AXIS2_PLACEMENT_3D('',#19741,#14907,#14908);
#11994=AXIS2_PLACEMENT_3D('',#19744,#14909,#14910);
#11995=AXIS2_PLACEMENT_3D('',#19748,#14912,#14913);
#11996=AXIS2_PLACEMENT_3D('',#19750,#14915,#14916);
#11997=AXIS2_PLACEMENT_3D('',#19756,#14920,#14921);
#11998=AXIS2_PLACEMENT_3D('',#19762,#14925,#14926);
#11999=AXIS2_PLACEMENT_3D('',#19763,#14927,#14928);
#12000=AXIS2_PLACEMENT_3D('',#19764,#14929,#14930);
#12001=AXIS2_PLACEMENT_3D('',#19765,#14931,#14932);
#12002=AXIS2_PLACEMENT_3D('',#19766,#14933,#14934);
#12003=AXIS2_PLACEMENT_3D('',#19767,#14935,#14936);
#12004=AXIS2_PLACEMENT_3D('',#19768,#14937,#14938);
#12005=AXIS2_PLACEMENT_3D('',#19770,#14940,#14941);
#12006=AXIS2_PLACEMENT_3D('',#19772,#14943,#14944);
#12007=AXIS2_PLACEMENT_3D('',#19774,#14946,#14947);
#12008=AXIS2_PLACEMENT_3D('',#19776,#14949,#14950);
#12009=AXIS2_PLACEMENT_3D('',#19777,#14951,#14952);
#14800=DIRECTION('axis',(0.,0.,1.));
#14801=DIRECTION('refdir',(1.,0.,0.));
#14802=DIRECTION('center_axis',(0.,1.,0.));
#14803=DIRECTION('ref_axis',(0.,0.,1.));
#14804=DIRECTION('center_axis',(6.93889390390722E-17,-1.,0.));
#14805=DIRECTION('ref_axis',(-1.,-6.93889390390722E-17,0.));
#14806=DIRECTION('',(0.,1.,0.));
#14807=DIRECTION('center_axis',(6.93889390390722E-17,1.,0.));
#14808=DIRECTION('ref_axis',(1.,-6.93889390390722E-17,0.));
#14809=DIRECTION('center_axis',(0.,1.,0.));
#14810=DIRECTION('ref_axis',(0.,0.,1.));
#14811=DIRECTION('center_axis',(0.,1.,0.));
#14812=DIRECTION('ref_axis',(0.,0.,1.));
#14813=DIRECTION('',(0.,1.,0.));
#14814=DIRECTION('center_axis',(0.,-1.,0.));
#14815=DIRECTION('ref_axis',(0.,0.,-1.));
#14816=DIRECTION('center_axis',(0.,1.,0.));
#14817=DIRECTION('ref_axis',(0.,0.,1.));
#14818=DIRECTION('center_axis',(0.,1.,0.));
#14819=DIRECTION('ref_axis',(0.,0.,1.));
#14820=DIRECTION('',(0.,1.,0.));
#14821=DIRECTION('center_axis',(0.,1.,0.));
#14822=DIRECTION('ref_axis',(0.,0.,1.));
#14823=DIRECTION('center_axis',(0.,1.,0.));
#14824=DIRECTION('ref_axis',(0.,0.,1.));
#14825=DIRECTION('center_axis',(0.,1.,0.));
#14826=DIRECTION('ref_axis',(0.,0.,1.));
#14827=DIRECTION('',(0.,1.,0.));
#14828=DIRECTION('center_axis',(0.,-1.,0.));
#14829=DIRECTION('ref_axis',(0.,0.,-1.));
#14830=DIRECTION('center_axis',(0.,1.,0.));
#14831=DIRECTION('ref_axis',(0.,0.,1.));
#14832=DIRECTION('center_axis',(0.,1.,0.));
#14833=DIRECTION('ref_axis',(0.,0.,1.));
#14834=DIRECTION('',(0.,1.,0.));
#14835=DIRECTION('center_axis',(0.,1.,0.));
#14836=DIRECTION('ref_axis',(0.,0.,1.));
#14837=DIRECTION('center_axis',(1.,0.,0.));
#14838=DIRECTION('ref_axis',(0.,0.,-1.));
#14839=DIRECTION('',(0.,0.,-1.));
#14840=DIRECTION('',(0.,1.,0.));
#14841=DIRECTION('',(0.,0.,-1.));
#14842=DIRECTION('',(0.,-1.,0.));
#14843=DIRECTION('center_axis',(0.,1.,0.));
#14844=DIRECTION('ref_axis',(0.,0.,1.));
#14845=DIRECTION('',(1.,0.,0.));
#14846=DIRECTION('',(-0.707106781186546,0.,-0.707106781186549));
#14847=DIRECTION('',(0.707106781186548,0.,-0.707106781186547));
#14848=DIRECTION('',(1.,0.,0.));
#14849=DIRECTION('',(0.,0.,-1.));
#14850=DIRECTION('center_axis',(1.,3.06127672231201E-16,0.));
#14851=DIRECTION('ref_axis',(-3.06127672231201E-16,1.,0.));
#14852=DIRECTION('',(3.06127672231201E-16,-1.,0.));
#14853=DIRECTION('',(0.,0.,-1.));
#14854=DIRECTION('',(3.06127672231201E-16,-1.,0.));
#14855=DIRECTION('center_axis',(0.,-1.,0.));
#14856=DIRECTION('ref_axis',(0.,0.,-1.));
#14857=DIRECTION('',(0.,0.,-1.));
#14858=DIRECTION('',(0.707106781186546,0.,0.707106781186549));
#14859=DIRECTION('',(-1.,0.,0.));
#14860=DIRECTION('',(-1.,0.,0.));
#14861=DIRECTION('',(-0.707106781186548,0.,0.707106781186547));
#14862=DIRECTION('center_axis',(1.,0.,0.));
#14863=DIRECTION('ref_axis',(0.,0.,-1.));
#14864=DIRECTION('',(0.,0.,-1.));
#14865=DIRECTION('',(0.,1.,0.));
#14866=DIRECTION('',(0.,-1.,0.));
#14867=DIRECTION('center_axis',(0.,1.,0.));
#14868=DIRECTION('ref_axis',(0.,0.,1.));
#14869=DIRECTION('',(1.,0.,0.));
#14870=DIRECTION('',(0.,0.,1.));
#14871=DIRECTION('',(1.,0.,0.));
#14872=DIRECTION('',(-0.707106781186546,0.,-0.707106781186549));
#14873=DIRECTION('',(0.707106781186548,0.,-0.707106781186547));
#14874=DIRECTION('center_axis',(0.,-1.,0.));
#14875=DIRECTION('ref_axis',(0.,0.,-1.));
#14876=DIRECTION('',(-1.,0.,0.));
#14877=DIRECTION('',(0.,0.,-1.));
#14878=DIRECTION('',(-1.,0.,0.));
#14879=DIRECTION('',(-0.707106781186548,0.,0.707106781186547));
#14880=DIRECTION('',(0.707106781186546,0.,0.707106781186549));
#14881=DIRECTION('center_axis',(0.,0.,1.));
#14882=DIRECTION('ref_axis',(1.,0.,0.));
#14883=DIRECTION('',(0.707106781186545,0.70710678118655,0.));
#14884=DIRECTION('',(0.,1.,0.));
#14885=DIRECTION('',(0.,1.,0.));
#14886=DIRECTION('',(-5.71424710475988E-16,-1.,0.));
#14887=DIRECTION('',(-0.707106781186549,0.707106781186546,0.));
#14888=DIRECTION('',(0.,-1.,0.));
#14889=DIRECTION('',(0.,-1.,0.));
#14890=DIRECTION('center_axis',(0.,0.,1.));
#14891=DIRECTION('ref_axis',(1.,0.,0.));
#14892=DIRECTION('',(0.,1.,0.));
#14893=DIRECTION('',(-0.707106781186545,-0.70710678118655,0.));
#14894=DIRECTION('',(0.,1.,0.));
#14895=DIRECTION('',(0.,1.,0.));
#14896=DIRECTION('',(0.707106781186549,-0.707106781186546,0.));
#14897=DIRECTION('',(-5.71424710475988E-16,-1.,0.));
#14898=DIRECTION('',(0.,1.,0.));
#14899=DIRECTION('center_axis',(-0.707106781186549,0.,0.707106781186546));
#14900=DIRECTION('ref_axis',(0.,1.,0.));
#14901=DIRECTION('center_axis',(0.707106781186547,0.,0.707106781186548));
#14902=DIRECTION('ref_axis',(0.,-1.,0.));
#14903=DIRECTION('center_axis',(-0.707106781186549,0.,0.707106781186546));
#14904=DIRECTION('ref_axis',(0.,1.,0.));
#14905=DIRECTION('center_axis',(0.707106781186547,0.,0.707106781186548));
#14906=DIRECTION('ref_axis',(0.,-1.,0.));
#14907=DIRECTION('center_axis',(0.,1.,0.));
#14908=DIRECTION('ref_axis',(0.,0.,1.));
#14909=DIRECTION('center_axis',(6.93889390390722E-17,-1.,0.));
#14910=DIRECTION('ref_axis',(-1.,-6.93889390390722E-17,0.));
#14911=DIRECTION('',(0.,1.,0.));
#14912=DIRECTION('center_axis',(6.93889390390722E-17,1.,0.));
#14913=DIRECTION('ref_axis',(1.,-6.93889390390723E-17,0.));
#14914=DIRECTION('',(0.,1.,0.));
#14915=DIRECTION('center_axis',(0.,0.,1.));
#14916=DIRECTION('ref_axis',(1.,0.,0.));
#14917=DIRECTION('',(-1.,-6.93889390390722E-17,0.));
#14918=DIRECTION('',(1.,-6.93889390390722E-17,0.));
#14919=DIRECTION('',(0.,-1.,0.));
#14920=DIRECTION('center_axis',(0.,0.,-1.));
#14921=DIRECTION('ref_axis',(-1.,0.,0.));
#14922=DIRECTION('',(1.,6.93889390390722E-17,0.));
#14923=DIRECTION('',(0.,1.,0.));
#14924=DIRECTION('',(-1.,6.93889390390722E-17,0.));
#14925=DIRECTION('center_axis',(0.,1.,0.));
#14926=DIRECTION('ref_axis',(0.,0.,1.));
#14927=DIRECTION('center_axis',(6.93889390390722E-17,-1.,0.));
#14928=DIRECTION('ref_axis',(-1.,-6.93889390390722E-17,8.67361737988404E-16));
#14929=DIRECTION('center_axis',(6.93889390390722E-17,1.,0.));
#14930=DIRECTION('ref_axis',(1.,-6.93889390390722E-17,0.));
#14931=DIRECTION('center_axis',(0.,1.,0.));
#14932=DIRECTION('ref_axis',(0.,0.,1.));
#14933=DIRECTION('center_axis',(6.93889390390722E-17,-1.,0.));
#14934=DIRECTION('ref_axis',(-1.,-6.93889390390722E-17,6.93889390390723E-16));
#14935=DIRECTION('center_axis',(6.93889390390722E-17,1.,0.));
#14936=DIRECTION('ref_axis',(1.,-6.93889390390722E-17,0.));
#14937=DIRECTION('center_axis',(-6.93889390390722E-17,-1.,0.));
#14938=DIRECTION('ref_axis',(1.,-6.93889390390723E-17,0.));
#14939=DIRECTION('',(0.,0.,1.));
#14940=DIRECTION('center_axis',(-1.,5.71424710475987E-16,0.));
#14941=DIRECTION('ref_axis',(-5.71424710475987E-16,-1.,0.));
#14942=DIRECTION('',(0.,0.,1.));
#14943=DIRECTION('center_axis',(-6.93889390390722E-17,1.,0.));
#14944=DIRECTION('ref_axis',(-1.,-6.93889390390723E-17,0.));
#14945=DIRECTION('',(0.,0.,1.));
#14946=DIRECTION('center_axis',(-1.,-5.71424710475987E-16,0.));
#14947=DIRECTION('ref_axis',(5.71424710475987E-16,-1.,0.));
#14948=DIRECTION('',(0.,0.,-1.));
#14949=DIRECTION('center_axis',(-0.70710678118655,0.707106781186545,0.));
#14950=DIRECTION('ref_axis',(0.,0.,1.));
#14951=DIRECTION('center_axis',(-0.707106781186546,-0.707106781186549,0.));
#14952=DIRECTION('ref_axis',(0.,0.,1.));
#19621=CARTESIAN_POINT('',(0.,0.,0.));
#19622=CARTESIAN_POINT('Origin',(13.,-20.,19.5));
#19623=CARTESIAN_POINT('',(13.,-10.,11.5));
#19624=CARTESIAN_POINT('Origin',(13.,-10.,19.5));
#19625=CARTESIAN_POINT('',(13.,10.,11.5));
#19626=CARTESIAN_POINT('',(13.,-20.,11.5));
#19627=CARTESIAN_POINT('Origin',(13.,10.,19.5));
#19628=CARTESIAN_POINT('Origin',(-7.7,-20.,25.5));
#19629=CARTESIAN_POINT('',(-7.7,-20.,24.25));
#19630=CARTESIAN_POINT('Origin',(-7.7,-20.,25.5));
#19631=CARTESIAN_POINT('',(-7.7,-17.,24.25));
#19632=CARTESIAN_POINT('',(-7.7,-20.,24.25));
#19633=CARTESIAN_POINT('Origin',(-7.7,-17.,25.5));
#19634=CARTESIAN_POINT('Origin',(-7.7,-20.,25.5));
#19635=CARTESIAN_POINT('',(-7.7,17.,24.25));
#19636=CARTESIAN_POINT('Origin',(-7.7,17.,25.5));
#19637=CARTESIAN_POINT('',(-7.7,20.,24.25));
#19638=CARTESIAN_POINT('',(-7.7,-20.,24.25));
#19639=CARTESIAN_POINT('Origin',(-7.7,20.,25.5));
#19640=CARTESIAN_POINT('Origin',(-7.7,-20.,3.5));
#19641=CARTESIAN_POINT('',(-7.7,-20.,2.25));
#19642=CARTESIAN_POINT('Origin',(-7.7,-20.,3.5));
#19643=CARTESIAN_POINT('',(-7.7,-17.,2.25));
#19644=CARTESIAN_POINT('',(-7.7,-20.,2.25));
#19645=CARTESIAN_POINT('Origin',(-7.7,-17.,3.5));
#19646=CARTESIAN_POINT('Origin',(-7.7,-20.,3.5));
#19647=CARTESIAN_POINT('',(-7.7,17.,2.25));
#19648=CARTESIAN_POINT('Origin',(-7.7,17.,3.5));
#19649=CARTESIAN_POINT('',(-7.7,20.,2.25));
#19650=CARTESIAN_POINT('',(-7.7,-20.,2.25));
#19651=CARTESIAN_POINT('Origin',(-7.7,20.,3.5));
#19652=CARTESIAN_POINT('Origin',(-10.5,20.,36.));
#19653=CARTESIAN_POINT('',(-10.5,17.,33.));
#19654=CARTESIAN_POINT('',(-10.5,17.,3.00000000000001));
#19655=CARTESIAN_POINT('',(-10.5,17.,36.));
#19656=CARTESIAN_POINT('',(-10.5,20.,33.));
#19657=CARTESIAN_POINT('',(-10.5,20.,33.));
#19658=CARTESIAN_POINT('',(-10.5,20.,3.00000000000001));
#19659=CARTESIAN_POINT('',(-10.5,20.,36.));
#19660=CARTESIAN_POINT('',(-10.5,20.,3.));
#19661=CARTESIAN_POINT('Origin',(-10.5,17.,36.));
#19662=CARTESIAN_POINT('',(-7.5,17.,36.));
#19663=CARTESIAN_POINT('',(-3.,17.,36.));
#19664=CARTESIAN_POINT('',(-10.5,17.,36.));
#19665=CARTESIAN_POINT('',(-7.5,17.,36.));
#19666=CARTESIAN_POINT('',(-7.49999999999999,17.,0.));
#19667=CARTESIAN_POINT('',(-10.5,17.,3.));
#19668=CARTESIAN_POINT('',(-3.,17.,0.));
#19669=CARTESIAN_POINT('',(-10.5,17.,0.));
#19670=CARTESIAN_POINT('',(-3.,17.,36.));
#19671=CARTESIAN_POINT('Origin',(-3.,17.,36.));
#19672=CARTESIAN_POINT('',(-2.99999999999999,-17.,0.));
#19673=CARTESIAN_POINT('',(-3.,17.,0.));
#19674=CARTESIAN_POINT('',(-2.99999999999999,-17.,36.));
#19675=CARTESIAN_POINT('',(-2.99999999999999,-17.,36.));
#19676=CARTESIAN_POINT('',(-3.,17.,36.));
#19677=CARTESIAN_POINT('Origin',(-10.5,-17.,36.));
#19678=CARTESIAN_POINT('',(-10.5,-17.,33.));
#19679=CARTESIAN_POINT('',(-10.5,-17.,3.00000000000001));
#19680=CARTESIAN_POINT('',(-10.5,-17.,36.));
#19681=CARTESIAN_POINT('',(-7.5,-17.,36.));
#19682=CARTESIAN_POINT('',(-7.5,-17.,36.));
#19683=CARTESIAN_POINT('',(-10.5,-17.,36.));
#19684=CARTESIAN_POINT('',(-7.49999999999999,-17.,-2.16840434497101E-16));
#19685=CARTESIAN_POINT('',(-10.5,-17.,0.));
#19686=CARTESIAN_POINT('',(-10.5,-17.,3.));
#19687=CARTESIAN_POINT('Origin',(-10.5,-17.,36.));
#19688=CARTESIAN_POINT('',(-10.5,-20.,33.));
#19689=CARTESIAN_POINT('',(-10.5,-20.,3.00000000000001));
#19690=CARTESIAN_POINT('',(-10.5,-20.,36.));
#19691=CARTESIAN_POINT('',(-10.5,-17.,33.));
#19692=CARTESIAN_POINT('',(-10.5,-17.,3.));
#19693=CARTESIAN_POINT('Origin',(-10.5,-20.,36.));
#19694=CARTESIAN_POINT('',(-7.49999999999999,-20.,0.));
#19695=CARTESIAN_POINT('',(-2.,-20.,0.));
#19696=CARTESIAN_POINT('',(-10.5,-20.,0.));
#19697=CARTESIAN_POINT('',(-2.,-20.,36.));
#19698=CARTESIAN_POINT('',(-2.,-20.,36.));
#19699=CARTESIAN_POINT('',(-7.5,-20.,36.));
#19700=CARTESIAN_POINT('',(-10.5,-20.,36.));
#19701=CARTESIAN_POINT('',(-7.5,-20.,36.));
#19702=CARTESIAN_POINT('',(-10.5,-20.,3.));
#19703=CARTESIAN_POINT('Origin',(-10.5,20.,36.));
#19704=CARTESIAN_POINT('',(-2.00000000000001,20.,36.));
#19705=CARTESIAN_POINT('',(-7.5,20.,36.));
#19706=CARTESIAN_POINT('',(-10.5,20.,36.));
#19707=CARTESIAN_POINT('',(-2.00000000000001,20.,0.));
#19708=CARTESIAN_POINT('',(-2.00000000000001,20.,36.));
#19709=CARTESIAN_POINT('',(-7.49999999999999,20.,-2.16840434497101E-16));
#19710=CARTESIAN_POINT('',(-10.5,20.,0.));
#19711=CARTESIAN_POINT('',(-10.5,20.,3.));
#19712=CARTESIAN_POINT('',(-7.5,20.,36.));
#19713=CARTESIAN_POINT('Origin',(0.,0.,36.));
#19714=CARTESIAN_POINT('',(6.93889390390723E-15,-18.,36.));
#19715=CARTESIAN_POINT('',(8.99999999999999,-8.99999999999993,36.));
#19716=CARTESIAN_POINT('',(6.93889390390723E-15,-10.,36.));
#19717=CARTESIAN_POINT('',(6.93889390390723E-15,20.,36.));
#19718=CARTESIAN_POINT('',(1.22464679914735E-15,10.,36.));
#19719=CARTESIAN_POINT('',(6.93889390390723E-15,20.,36.));
#19720=CARTESIAN_POINT('',(5.50010745544284E-15,18.,36.));
#19721=CARTESIAN_POINT('',(6.93889390390723E-15,20.,36.));
#19722=CARTESIAN_POINT('',(9.,9.00000000000003,36.));
#19723=CARTESIAN_POINT('',(-7.5,17.,36.));
#19724=CARTESIAN_POINT('',(-7.5,-20.,36.));
#19725=CARTESIAN_POINT('Origin',(0.,0.,0.));
#19726=CARTESIAN_POINT('',(6.50521303491303E-15,-18.,0.));
#19727=CARTESIAN_POINT('',(1.22464679914735E-15,-10.,0.));
#19728=CARTESIAN_POINT('',(6.93889390390723E-15,20.,0.));
#19729=CARTESIAN_POINT('',(-2.,-20.,0.));
#19730=CARTESIAN_POINT('',(-7.49999999999999,0.,0.));
#19731=CARTESIAN_POINT('',(-7.49999999999999,0.,0.));
#19732=CARTESIAN_POINT('',(5.79604448295525E-15,18.,0.));
#19733=CARTESIAN_POINT('',(5.79604448295525E-15,18.,0.));
#19734=CARTESIAN_POINT('',(1.22464679914735E-15,10.,0.));
#19735=CARTESIAN_POINT('',(6.93889390390723E-15,20.,0.));
#19736=CARTESIAN_POINT('',(6.93889390390723E-15,20.,0.));
#19737=CARTESIAN_POINT('Origin',(-7.5,0.,36.));
#19738=CARTESIAN_POINT('Origin',(-10.5,-17.,3.));
#19739=CARTESIAN_POINT('Origin',(-7.5,0.,36.));
#19740=CARTESIAN_POINT('Origin',(-10.5,20.,3.));
#19741=CARTESIAN_POINT('Origin',(13.,-20.,19.5));
#19742=CARTESIAN_POINT('',(13.,-10.,7.5));
#19743=CARTESIAN_POINT('',(13.,-10.,31.5));
#19744=CARTESIAN_POINT('Origin',(13.,-10.,19.5));
#19745=CARTESIAN_POINT('',(13.,10.,7.5));
#19746=CARTESIAN_POINT('',(13.,-20.,7.5));
#19747=CARTESIAN_POINT('',(13.,10.,31.5));
#19748=CARTESIAN_POINT('Origin',(13.,10.,19.5));
#19749=CARTESIAN_POINT('',(13.,-20.,31.5));
#19750=CARTESIAN_POINT('Origin',(13.,-20.,31.5));
#19751=CARTESIAN_POINT('',(8.35164654424504,-10.,31.5));
#19752=CARTESIAN_POINT('',(13.,-10.,31.5));
#19753=CARTESIAN_POINT('',(8.35164654424504,10.,31.5));
#19754=CARTESIAN_POINT('',(13.,10.,31.5));
#19755=CARTESIAN_POINT('',(8.35164654424504,-20.,31.5));
#19756=CARTESIAN_POINT('Origin',(13.,-20.,7.5));
#19757=CARTESIAN_POINT('',(9.68245836551855,-10.,7.5));
#19758=CARTESIAN_POINT('',(13.,-10.,7.5));
#19759=CARTESIAN_POINT('',(9.68245836551855,10.,7.5));
#19760=CARTESIAN_POINT('',(9.68245836551855,20.,7.5));
#19761=CARTESIAN_POINT('',(13.,10.,7.5));
#19762=CARTESIAN_POINT('Origin',(9.68245836551855,20.,-2.5));
#19763=CARTESIAN_POINT('Origin',(9.68245836551855,-10.,-2.5));
#19764=CARTESIAN_POINT('Origin',(9.68245836551855,10.,-2.5));
#19765=CARTESIAN_POINT('Origin',(8.35164654424504,20.,41.5));
#19766=CARTESIAN_POINT('Origin',(8.35164654424504,-10.,41.5));
#19767=CARTESIAN_POINT('Origin',(8.35164654424504,10.,41.5));
#19768=CARTESIAN_POINT('Origin',(1.22464679914735E-15,10.,0.));
#19769=CARTESIAN_POINT('',(1.22464679914735E-15,10.,0.));
#19770=CARTESIAN_POINT('Origin',(6.93889390390723E-15,20.,0.));
#19771=CARTESIAN_POINT('',(5.79604448295525E-15,18.,0.));
#19772=CARTESIAN_POINT('Origin',(1.22464679914735E-15,-10.,0.));
#19773=CARTESIAN_POINT('',(1.22464679914735E-15,-10.,0.));
#19774=CARTESIAN_POINT('Origin',(6.93889390390723E-15,-20.,0.));
#19775=CARTESIAN_POINT('',(5.79604448295524E-15,-18.,0.));
#19776=CARTESIAN_POINT('Origin',(-2.,-20.,36.));
#19777=CARTESIAN_POINT('Origin',(5.79604448295525E-15,18.,0.));
#20154=UNCERTAINTY_MEASURE_WITH_UNIT(LENGTH_MEASURE(0.01),#20177,
'DISTANCE_ACCURACY_VALUE',
'Maximum model space distance between geometric entities at asserted c
onnectivities');
#20160=UNCERTAINTY_MEASURE_WITH_UNIT(LENGTH_MEASURE(0.01),#20177,
'DISTANCE_ACCURACY_VALUE',
'Maximum model space distance between geometric entities at asserted c
onnectivities');
#20170=(
GEOMETRIC_REPRESENTATION_CONTEXT(3)
GLOBAL_UNCERTAINTY_ASSIGNED_CONTEXT((#20154))
GLOBAL_UNIT_ASSIGNED_CONTEXT((#20177,#20179,#20180))
REPRESENTATION_CONTEXT('','3D')
);
#20176=(
GEOMETRIC_REPRESENTATION_CONTEXT(3)
GLOBAL_UNCERTAINTY_ASSIGNED_CONTEXT((#20160))
GLOBAL_UNIT_ASSIGNED_CONTEXT((#20177,#20179,#20180))
REPRESENTATION_CONTEXT('','3D')
);
#20177=(
LENGTH_UNIT()
NAMED_UNIT(*)
SI_UNIT(.MILLI.,.METRE.)
);
#20179=(
NAMED_UNIT(*)
PLANE_ANGLE_UNIT()
SI_UNIT($,.RADIAN.)
);
#20180=(
NAMED_UNIT(*)
SI_UNIT($,.STERADIAN.)
SOLID_ANGLE_UNIT()
);
#20190=SHAPE_DEFINITION_REPRESENTATION(#20205,#20264);
#20205=PRODUCT_DEFINITION_SHAPE('',$,#20280);
#20264=SHAPE_REPRESENTATION('',(#11964),#20170);
#20270=PRODUCT_DEFINITION_CONTEXT('part definition',#20317,'design');
#20280=PRODUCT_DEFINITION('Bearing Seat Bracket','Bearing Seat Bracket',
#20295,#20270);
#20295=PRODUCT_DEFINITION_FORMATION('',$,#20328);
#20317=APPLICATION_CONTEXT(
'Core Data for Automotive Mechanical Design Process');
#20318=PRODUCT_CONTEXT('part definition',#20317,'mechanical');
#20328=PRODUCT('Bearing Seat Bracket','Bearing Seat Bracket',$,(#20318));
#20338=PRESENTATION_STYLE_ASSIGNMENT((#20343));
#20343=SURFACE_STYLE_USAGE(.BOTH.,#20348);
#20348=SURFACE_SIDE_STYLE('',(#20353));
#20353=SURFACE_STYLE_FILL_AREA(#20358);
#20358=FILL_AREA_STYLE('Opaque(122,133,145)',(#20363));
#20363=FILL_AREA_STYLE_COLOUR('Opaque(122,133,145)',#20368);
#20368=COLOUR_RGB('Opaque(122,133,145)',0.47843137254902,0.52156862745098,
0.568627450980392);
ENDSEC;
END-ISO-10303-21;
